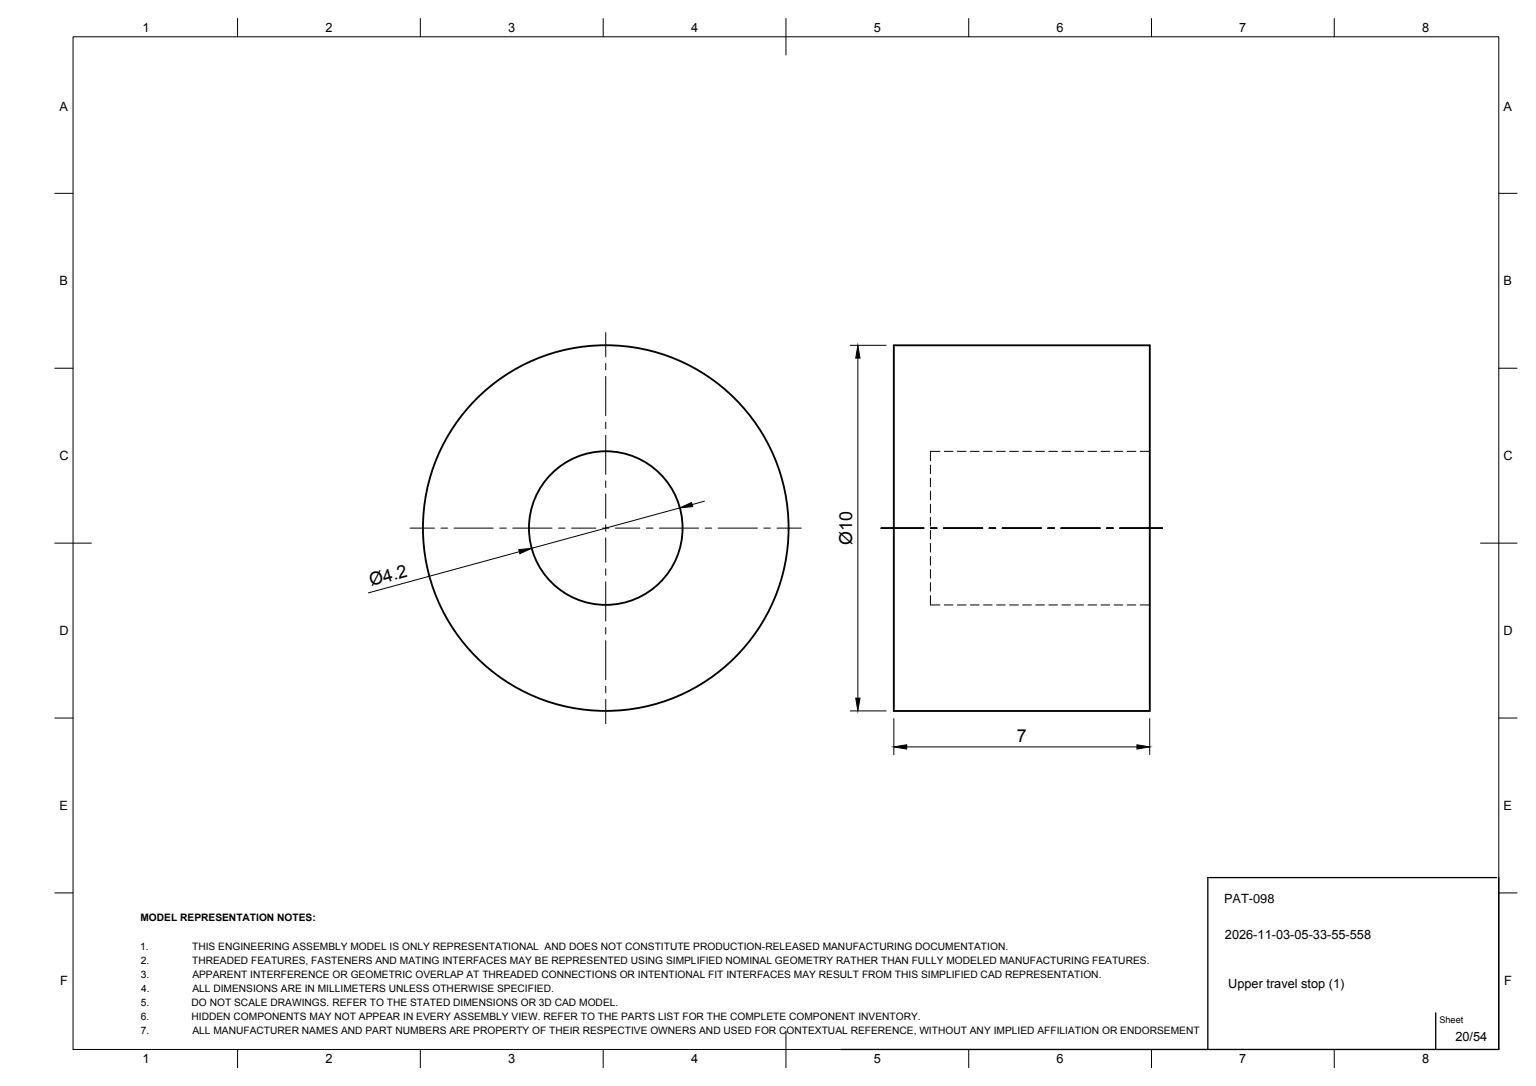
ISO-10303-21;
HEADER;
/* Generated by software containing ST-Developer
 * from STEP Tools, Inc. (www.steptools.com) 
 */

FILE_DESCRIPTION(
/* description */ ('Spring compression tester'),
/* implementation_level */ '2;1');

FILE_NAME(
/* name */ 'Upper travel stop (1).step',
/* time_stamp */ '2026-10-28T03:24:11-07:00',
/* author */ (''),
/* organization */ (''),
/* preprocessor_version */ 'ST-DEVELOPER v20.2',
/* originating_system */ 'Autodesk Translation Framework v15.17.0.0',
/* authorisation */ '');

FILE_SCHEMA (('AUTOMOTIVE_DESIGN { 1 0 10303 214 3 1 1 }'));
ENDSEC;

DATA;
#10=MECHANICAL_DESIGN_GEOMETRIC_PRESENTATION_REPRESENTATION('',(#1121),#43521);
#1001=SHAPE_REPRESENTATION_RELATIONSHIP('SRR','None',#43813,#1061);
#1061=ADVANCED_BREP_SHAPE_REPRESENTATION('',(#1196),#43473);
#1121=STYLED_ITEM('',(#44216),#1196);
#1196=MANIFOLD_SOLID_BREP('Body1',#18558);
#1397=FACE_BOUND('',#3600,.T.);
#1719=PLANE('',#19742);
#1720=PLANE('',#19746);
#1721=PLANE('',#19747);
#2399=FACE_OUTER_BOUND('',#3596,.T.);
#2400=FACE_OUTER_BOUND('',#3597,.T.);
#2401=FACE_OUTER_BOUND('',#3598,.T.);
#2402=FACE_OUTER_BOUND('',#3599,.T.);
#2403=FACE_OUTER_BOUND('',#3601,.T.);
#3596=EDGE_LOOP('',(#13219,#13220,#13221,#13222));
#3597=EDGE_LOOP('',(#13223));
#3598=EDGE_LOOP('',(#13224,#13225,#13226,#13227));
#3599=EDGE_LOOP('',(#13228));
#3600=EDGE_LOOP('',(#13229));
#3601=EDGE_LOOP('',(#13230));
#4901=LINE('',#27540,#6333);
#4902=LINE('',#27547,#6334);
#6333=VECTOR('',#22405,0.21);
#6334=VECTOR('',#22414,0.5);
#7676=CIRCLE('',#19740,0.21);
#7677=CIRCLE('',#19741,0.21);
#7678=CIRCLE('',#19744,0.5);
#7679=CIRCLE('',#19745,0.5);
#8470=VERTEX_POINT('',#27537);
#8471=VERTEX_POINT('',#27539);
#8472=VERTEX_POINT('',#27544);
#8473=VERTEX_POINT('',#27546);
#10274=EDGE_CURVE('',#8470,#8470,#7676,.T.);
#10275=EDGE_CURVE('',#8470,#8471,#4901,.T.);
#10276=EDGE_CURVE('',#8471,#8471,#7677,.T.);
#10277=EDGE_CURVE('',#8472,#8472,#7678,.T.);
#10278=EDGE_CURVE('',#8472,#8473,#4902,.T.);
#10279=EDGE_CURVE('',#8473,#8473,#7679,.T.);
#13219=ORIENTED_EDGE('',*,*,#10274,.F.);
#13220=ORIENTED_EDGE('',*,*,#10275,.T.);
#13221=ORIENTED_EDGE('',*,*,#10276,.F.);
#13222=ORIENTED_EDGE('',*,*,#10275,.F.);
#13223=ORIENTED_EDGE('',*,*,#10274,.T.);
#13224=ORIENTED_EDGE('',*,*,#10277,.F.);
#13225=ORIENTED_EDGE('',*,*,#10278,.T.);
#13226=ORIENTED_EDGE('',*,*,#10279,.T.);
#13227=ORIENTED_EDGE('',*,*,#10278,.F.);
#13228=ORIENTED_EDGE('',*,*,#10277,.T.);
#13229=ORIENTED_EDGE('',*,*,#10276,.T.);
#13230=ORIENTED_EDGE('',*,*,#10279,.F.);
#17204=CYLINDRICAL_SURFACE('',#19739,0.21);
#17205=CYLINDRICAL_SURFACE('',#19743,0.5);
#17723=ADVANCED_FACE('',(#2399),#17204,.F.);
#17724=ADVANCED_FACE('',(#2400),#1719,.T.);
#17725=ADVANCED_FACE('',(#2401),#17205,.T.);
#17726=ADVANCED_FACE('',(#2402,#1397),#1720,.T.);
#17727=ADVANCED_FACE('',(#2403),#1721,.F.);
#18558=CLOSED_SHELL('',(#17723,#17724,#17725,#17726,#17727));
#19738=AXIS2_PLACEMENT_3D('',#27535,#22399,#22400);
#19739=AXIS2_PLACEMENT_3D('',#27536,#22401,#22402);
#19740=AXIS2_PLACEMENT_3D('',#27538,#22403,#22404);
#19741=AXIS2_PLACEMENT_3D('',#27541,#22406,#22407);
#19742=AXIS2_PLACEMENT_3D('',#27542,#22408,#22409);
#19743=AXIS2_PLACEMENT_3D('',#27543,#22410,#22411);
#19744=AXIS2_PLACEMENT_3D('',#27545,#22412,#22413);
#19745=AXIS2_PLACEMENT_3D('',#27548,#22415,#22416);
#19746=AXIS2_PLACEMENT_3D('',#27549,#22417,#22418);
#19747=AXIS2_PLACEMENT_3D('',#27550,#22419,#22420);
#22399=DIRECTION('axis',(0.,0.,1.));
#22400=DIRECTION('refdir',(1.,0.,0.));
#22401=DIRECTION('center_axis',(0.,0.,1.));
#22402=DIRECTION('ref_axis',(1.,0.,0.));
#22403=DIRECTION('center_axis',(0.,0.,1.));
#22404=DIRECTION('ref_axis',(1.,0.,0.));
#22405=DIRECTION('',(0.,0.,1.));
#22406=DIRECTION('center_axis',(0.,0.,-1.));
#22407=DIRECTION('ref_axis',(1.,0.,0.));
#22408=DIRECTION('center_axis',(0.,0.,1.));
#22409=DIRECTION('ref_axis',(1.,0.,0.));
#22410=DIRECTION('center_axis',(0.,0.,1.));
#22411=DIRECTION('ref_axis',(1.,0.,0.));
#22412=DIRECTION('center_axis',(0.,0.,1.));
#22413=DIRECTION('ref_axis',(1.,0.,0.));
#22414=DIRECTION('',(0.,0.,-1.));
#22415=DIRECTION('center_axis',(0.,0.,1.));
#22416=DIRECTION('ref_axis',(1.,0.,0.));
#22417=DIRECTION('center_axis',(0.,0.,1.));
#22418=DIRECTION('ref_axis',(1.,0.,0.));
#22419=DIRECTION('center_axis',(0.,0.,1.));
#22420=DIRECTION('ref_axis',(1.,0.,0.));
#27535=CARTESIAN_POINT('',(0.,0.,0.));
#27536=CARTESIAN_POINT('Origin',(6.,5.,22.4));
#27537=CARTESIAN_POINT('',(5.79,5.,22.4));
#27538=CARTESIAN_POINT('Origin',(6.,5.,22.4));
#27539=CARTESIAN_POINT('',(5.79,5.,23.));
#27540=CARTESIAN_POINT('',(5.79,5.,22.4));
#27541=CARTESIAN_POINT('Origin',(6.,5.,23.));
#27542=CARTESIAN_POINT('Origin',(6.,5.,22.4));
#27543=CARTESIAN_POINT('Origin',(6.,5.,22.3));
#27544=CARTESIAN_POINT('',(5.5,5.,23.));
#27545=CARTESIAN_POINT('Origin',(6.,5.,23.));
#27546=CARTESIAN_POINT('',(5.5,5.,22.3));
#27547=CARTESIAN_POINT('',(5.5,5.,22.3));
#27548=CARTESIAN_POINT('Origin',(6.,5.,22.3));
#27549=CARTESIAN_POINT('Origin',(6.,5.,23.));
#27550=CARTESIAN_POINT('Origin',(6.,5.,22.3));
#43405=UNCERTAINTY_MEASURE_WITH_UNIT(LENGTH_MEASURE(0.001),#43522,
'DISTANCE_ACCURACY_VALUE',
'Maximum model space distance between geometric entities at asserted c
onnectivities');
#43453=UNCERTAINTY_MEASURE_WITH_UNIT(LENGTH_MEASURE(0.001),#43522,
'DISTANCE_ACCURACY_VALUE',
'Maximum model space distance between geometric entities at asserted c
onnectivities');
#43473=(
GEOMETRIC_REPRESENTATION_CONTEXT(3)
GLOBAL_UNCERTAINTY_ASSIGNED_CONTEXT((#43405))
GLOBAL_UNIT_ASSIGNED_CONTEXT((#43522,#43524,#43525))
REPRESENTATION_CONTEXT('','3D')
);
#43521=(
GEOMETRIC_REPRESENTATION_CONTEXT(3)
GLOBAL_UNCERTAINTY_ASSIGNED_CONTEXT((#43453))
GLOBAL_UNIT_ASSIGNED_CONTEXT((#43522,#43524,#43525))
REPRESENTATION_CONTEXT('','3D')
);
#43522=(
LENGTH_UNIT()
NAMED_UNIT(*)
SI_UNIT(.CENTI.,.METRE.)
);
#43524=(
NAMED_UNIT(*)
PLANE_ANGLE_UNIT()
SI_UNIT($,.RADIAN.)
);
#43525=(
NAMED_UNIT(*)
SI_UNIT($,.STERADIAN.)
SOLID_ANGLE_UNIT()
);
#43545=SHAPE_DEFINITION_REPRESENTATION(#43612,#43813);
#43612=PRODUCT_DEFINITION_SHAPE('',$,#43881);
#43813=SHAPE_REPRESENTATION('',(#19738),#43473);
#43861=PRODUCT_DEFINITION_CONTEXT('part definition',#44064,'design');
#43881=PRODUCT_DEFINITION('Upper travel stop (1)','Upper travel stop (1)',
#43948,#43861);
#43948=PRODUCT_DEFINITION_FORMATION('',$,#44085);
#44064=APPLICATION_CONTEXT(
'Core Data for Automotive Mechanical Design Process');
#44065=PRODUCT_CONTEXT('part definition',#44064,'mechanical');
#44085=PRODUCT('Upper travel stop (1)','Upper travel stop (1)',
'Upper travel stop (1)',(#44065));
#44210=COLOUR_RGB('Off White',0.89,0.88,0.83);
#44211=FILL_AREA_STYLE_COLOUR('',#44210);
#44212=FILL_AREA_STYLE('',(#44211));
#44213=SURFACE_STYLE_FILL_AREA(#44212);
#44214=SURFACE_SIDE_STYLE('',(#44213));
#44215=SURFACE_STYLE_USAGE(.BOTH.,#44214);
#44216=PRESENTATION_STYLE_ASSIGNMENT((#44215));
ENDSEC;
END-ISO-10303-21;
